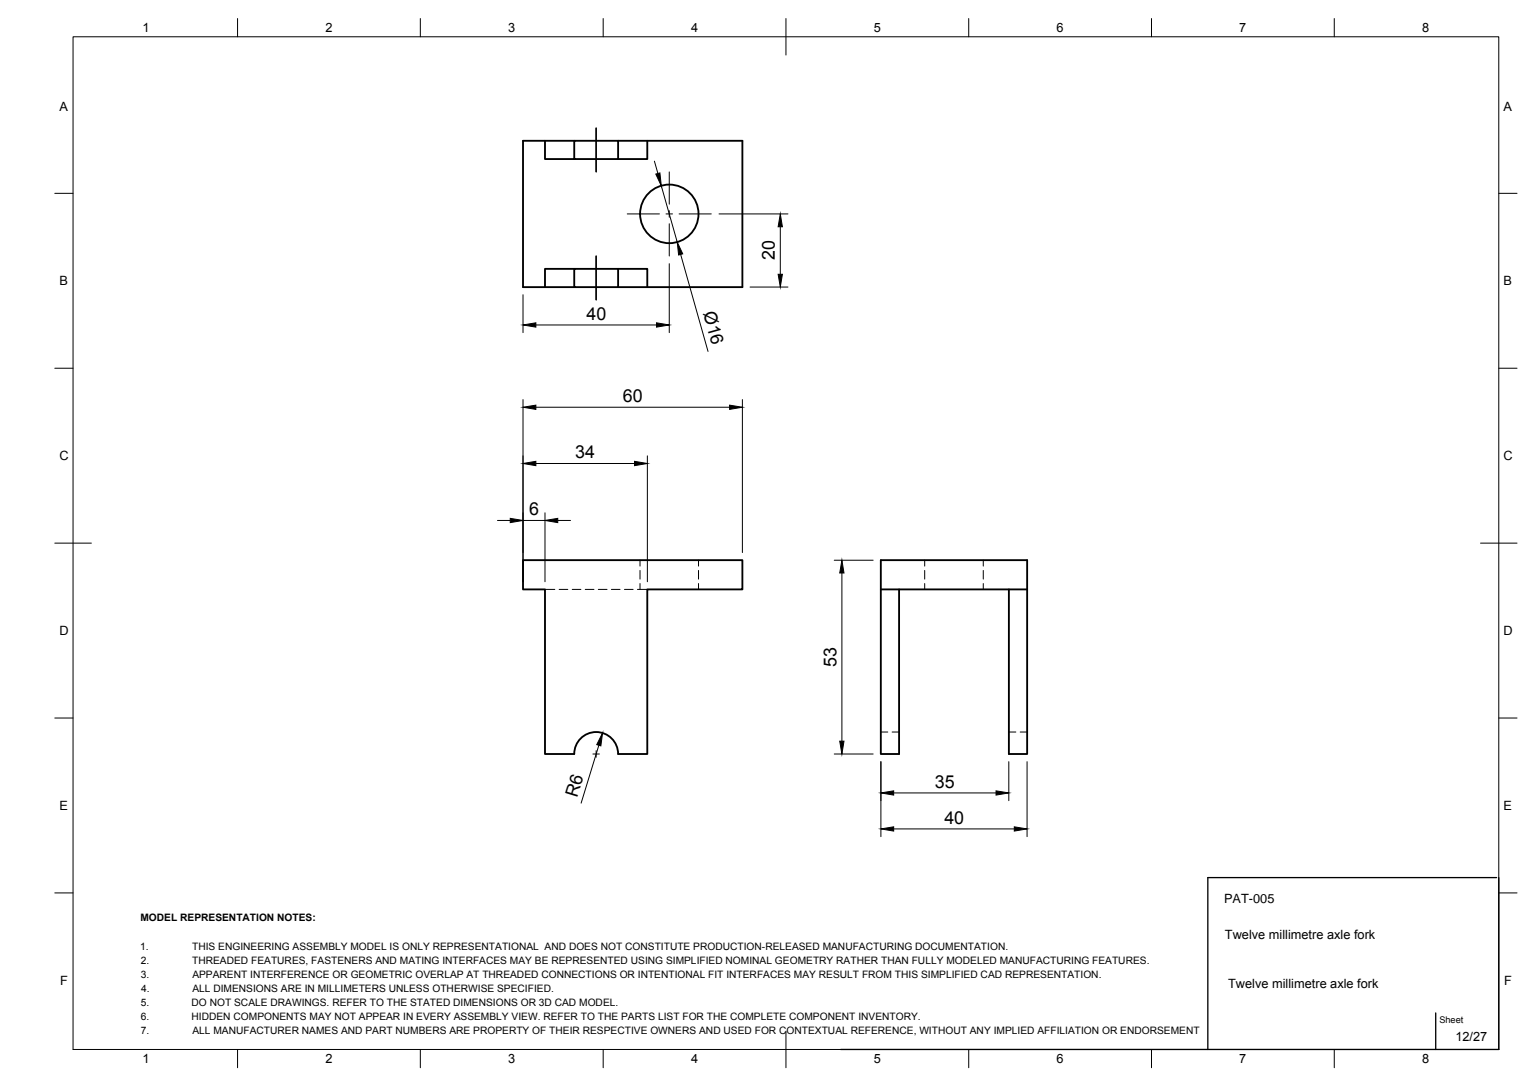
ISO-10303-21;
HEADER;
/* Generated by software containing ST-Developer
 * from STEP Tools, Inc. (www.steptools.com) 
 */

FILE_DESCRIPTION(
/* description */ ('Ball-race swivel caster'),
/* implementation_level */ '2;1');

FILE_NAME(
/* name */ 'Twelve millimetre axle fork.step',
/* time_stamp */ '2026-10-29T16:15:51-07:00',
/* author */ (''),
/* organization */ (''),
/* preprocessor_version */ 'ST-DEVELOPER v20.2',
/* originating_system */ 'Autodesk Translation Framework v15.17.0.0',
/* authorisation */ '');

FILE_SCHEMA (('AUTOMOTIVE_DESIGN { 1 0 10303 214 3 1 1 }'));
ENDSEC;

DATA;
#10=MECHANICAL_DESIGN_GEOMETRIC_PRESENTATION_REPRESENTATION('',(#314),#7816);
#265=SHAPE_REPRESENTATION_RELATIONSHIP('SRR','None',#7912,#285);
#285=ADVANCED_BREP_SHAPE_REPRESENTATION('',(#350),#7801);
#314=STYLED_ITEM('',(#8097),#350);
#350=MANIFOLD_SOLID_BREP('Body1',#3720);
#412=FACE_BOUND('',#883,.T.);
#413=FACE_BOUND('',#891,.T.);
#465=PLANE('',#4238);
#466=PLANE('',#4239);
#467=PLANE('',#4240);
#468=PLANE('',#4241);
#469=PLANE('',#4242);
#470=PLANE('',#4243);
#471=PLANE('',#4244);
#472=PLANE('',#4245);
#473=PLANE('',#4246);
#474=PLANE('',#4247);
#475=PLANE('',#4248);
#476=PLANE('',#4249);
#477=PLANE('',#4250);
#478=PLANE('',#4251);
#479=PLANE('',#4252);
#480=PLANE('',#4253);
#619=FACE_OUTER_BOUND('',#871,.T.);
#620=FACE_OUTER_BOUND('',#872,.T.);
#621=FACE_OUTER_BOUND('',#873,.T.);
#622=FACE_OUTER_BOUND('',#874,.T.);
#623=FACE_OUTER_BOUND('',#875,.T.);
#624=FACE_OUTER_BOUND('',#876,.T.);
#625=FACE_OUTER_BOUND('',#877,.T.);
#626=FACE_OUTER_BOUND('',#878,.T.);
#627=FACE_OUTER_BOUND('',#879,.T.);
#628=FACE_OUTER_BOUND('',#880,.T.);
#629=FACE_OUTER_BOUND('',#881,.T.);
#630=FACE_OUTER_BOUND('',#882,.T.);
#631=FACE_OUTER_BOUND('',#884,.T.);
#632=FACE_OUTER_BOUND('',#885,.T.);
#633=FACE_OUTER_BOUND('',#886,.T.);
#634=FACE_OUTER_BOUND('',#887,.T.);
#635=FACE_OUTER_BOUND('',#888,.T.);
#636=FACE_OUTER_BOUND('',#889,.T.);
#637=FACE_OUTER_BOUND('',#890,.T.);
#871=EDGE_LOOP('',(#2977,#2978,#2979,#2980));
#872=EDGE_LOOP('',(#2981,#2982,#2983,#2984));
#873=EDGE_LOOP('',(#2985,#2986,#2987,#2988));
#874=EDGE_LOOP('',(#2989,#2990,#2991,#2992,#2993,#2994,#2995,#2996,#2997,
#2998));
#875=EDGE_LOOP('',(#2999,#3000,#3001,#3002));
#876=EDGE_LOOP('',(#3003,#3004,#3005,#3006));
#877=EDGE_LOOP('',(#3007,#3008,#3009,#3010,#3011,#3012,#3013,#3014,#3015,
#3016));
#878=EDGE_LOOP('',(#3017,#3018,#3019,#3020));
#879=EDGE_LOOP('',(#3021,#3022,#3023,#3024));
#880=EDGE_LOOP('',(#3025,#3026,#3027,#3028));
#881=EDGE_LOOP('',(#3029,#3030,#3031,#3032,#3033,#3034));
#882=EDGE_LOOP('',(#3035,#3036,#3037,#3038,#3039,#3040,#3041,#3042,#3043,
#3044,#3045,#3046));
#883=EDGE_LOOP('',(#3047));
#884=EDGE_LOOP('',(#3048,#3049,#3050,#3051,#3052,#3053));
#885=EDGE_LOOP('',(#3054,#3055,#3056,#3057));
#886=EDGE_LOOP('',(#3058,#3059,#3060,#3061));
#887=EDGE_LOOP('',(#3062,#3063,#3064,#3065));
#888=EDGE_LOOP('',(#3066,#3067,#3068,#3069));
#889=EDGE_LOOP('',(#3070,#3071,#3072,#3073));
#890=EDGE_LOOP('',(#3074,#3075,#3076,#3077));
#891=EDGE_LOOP('',(#3078));
#1067=LINE('',#6943,#1222);
#1068=LINE('',#6950,#1223);
#1069=LINE('',#6953,#1224);
#1070=LINE('',#6957,#1225);
#1071=LINE('',#6961,#1226);
#1072=LINE('',#6965,#1227);
#1073=LINE('',#6967,#1228);
#1074=LINE('',#6969,#1229);
#1075=LINE('',#6971,#1230);
#1076=LINE('',#6973,#1231);
#1077=LINE('',#6975,#1232);
#1078=LINE('',#6977,#1233);
#1079=LINE('',#6979,#1234);
#1080=LINE('',#6980,#1235);
#1081=LINE('',#6983,#1236);
#1082=LINE('',#6984,#1237);
#1083=LINE('',#6987,#1238);
#1084=LINE('',#6988,#1239);
#1085=LINE('',#6991,#1240);
#1086=LINE('',#6993,#1241);
#1087=LINE('',#6995,#1242);
#1088=LINE('',#6997,#1243);
#1089=LINE('',#6999,#1244);
#1090=LINE('',#7001,#1245);
#1091=LINE('',#7003,#1246);
#1092=LINE('',#7005,#1247);
#1093=LINE('',#7006,#1248);
#1094=LINE('',#7009,#1249);
#1095=LINE('',#7010,#1250);
#1096=LINE('',#7013,#1251);
#1097=LINE('',#7014,#1252);
#1098=LINE('',#7017,#1253);
#1099=LINE('',#7018,#1254);
#1100=LINE('',#7020,#1255);
#1101=LINE('',#7022,#1256);
#1102=LINE('',#7024,#1257);
#1103=LINE('',#7026,#1258);
#1104=LINE('',#7027,#1259);
#1105=LINE('',#7028,#1260);
#1106=LINE('',#7031,#1261);
#1107=LINE('',#7032,#1262);
#1108=LINE('',#7033,#1263);
#1109=LINE('',#7036,#1264);
#1110=LINE('',#7039,#1265);
#1111=LINE('',#7041,#1266);
#1222=VECTOR('',#5083,0.8);
#1223=VECTOR('',#5090,1.);
#1224=VECTOR('',#5093,1.);
#1225=VECTOR('',#5096,1.);
#1226=VECTOR('',#5099,1.);
#1227=VECTOR('',#5104,1.);
#1228=VECTOR('',#5105,1.);
#1229=VECTOR('',#5106,1.);
#1230=VECTOR('',#5107,1.);
#1231=VECTOR('',#5108,1.);
#1232=VECTOR('',#5109,1.);
#1233=VECTOR('',#5110,1.);
#1234=VECTOR('',#5111,1.);
#1235=VECTOR('',#5112,1.);
#1236=VECTOR('',#5115,1.);
#1237=VECTOR('',#5116,1.);
#1238=VECTOR('',#5119,1.);
#1239=VECTOR('',#5120,1.);
#1240=VECTOR('',#5123,1.);
#1241=VECTOR('',#5124,1.);
#1242=VECTOR('',#5125,1.);
#1243=VECTOR('',#5126,1.);
#1244=VECTOR('',#5127,1.);
#1245=VECTOR('',#5128,1.);
#1246=VECTOR('',#5129,1.);
#1247=VECTOR('',#5130,1.);
#1248=VECTOR('',#5131,1.);
#1249=VECTOR('',#5134,1.);
#1250=VECTOR('',#5135,1.);
#1251=VECTOR('',#5138,1.);
#1252=VECTOR('',#5139,1.);
#1253=VECTOR('',#5142,1.);
#1254=VECTOR('',#5143,1.);
#1255=VECTOR('',#5146,1.);
#1256=VECTOR('',#5149,1.);
#1257=VECTOR('',#5150,1.);
#1258=VECTOR('',#5151,1.);
#1259=VECTOR('',#5152,1.);
#1260=VECTOR('',#5153,1.);
#1261=VECTOR('',#5156,1.);
#1262=VECTOR('',#5157,1.);
#1263=VECTOR('',#5158,1.);
#1264=VECTOR('',#5163,1.);
#1265=VECTOR('',#5168,1.);
#1266=VECTOR('',#5171,1.);
#1473=CIRCLE('',#4230,0.8);
#1474=CIRCLE('',#4231,0.8);
#1475=CIRCLE('',#4233,0.6);
#1476=CIRCLE('',#4234,0.6);
#1477=CIRCLE('',#4236,0.6);
#1478=CIRCLE('',#4237,0.6);
#1779=VERTEX_POINT('',#6940);
#1780=VERTEX_POINT('',#6942);
#1781=VERTEX_POINT('',#6946);
#1782=VERTEX_POINT('',#6947);
#1783=VERTEX_POINT('',#6949);
#1784=VERTEX_POINT('',#6951);
#1785=VERTEX_POINT('',#6955);
#1786=VERTEX_POINT('',#6956);
#1787=VERTEX_POINT('',#6958);
#1788=VERTEX_POINT('',#6960);
#1789=VERTEX_POINT('',#6964);
#1790=VERTEX_POINT('',#6966);
#1791=VERTEX_POINT('',#6968);
#1792=VERTEX_POINT('',#6970);
#1793=VERTEX_POINT('',#6972);
#1794=VERTEX_POINT('',#6974);
#1795=VERTEX_POINT('',#6976);
#1796=VERTEX_POINT('',#6978);
#1797=VERTEX_POINT('',#6982);
#1798=VERTEX_POINT('',#6986);
#1799=VERTEX_POINT('',#6990);
#1800=VERTEX_POINT('',#6992);
#1801=VERTEX_POINT('',#6994);
#1802=VERTEX_POINT('',#6996);
#1803=VERTEX_POINT('',#6998);
#1804=VERTEX_POINT('',#7000);
#1805=VERTEX_POINT('',#7002);
#1806=VERTEX_POINT('',#7004);
#1807=VERTEX_POINT('',#7008);
#1808=VERTEX_POINT('',#7012);
#1809=VERTEX_POINT('',#7016);
#1810=VERTEX_POINT('',#7023);
#1811=VERTEX_POINT('',#7025);
#1812=VERTEX_POINT('',#7030);
#2208=EDGE_CURVE('',#1779,#1779,#1473,.T.);
#2209=EDGE_CURVE('',#1779,#1780,#1067,.T.);
#2210=EDGE_CURVE('',#1780,#1780,#1474,.T.);
#2211=EDGE_CURVE('',#1781,#1782,#1475,.T.);
#2212=EDGE_CURVE('',#1783,#1781,#1068,.T.);
#2213=EDGE_CURVE('',#1784,#1783,#1476,.T.);
#2214=EDGE_CURVE('',#1782,#1784,#1069,.T.);
#2215=EDGE_CURVE('',#1785,#1786,#1070,.T.);
#2216=EDGE_CURVE('',#1787,#1785,#1477,.T.);
#2217=EDGE_CURVE('',#1788,#1787,#1071,.T.);
#2218=EDGE_CURVE('',#1786,#1788,#1478,.T.);
#2219=EDGE_CURVE('',#1785,#1789,#1072,.T.);
#2220=EDGE_CURVE('',#1789,#1790,#1073,.T.);
#2221=EDGE_CURVE('',#1790,#1791,#1074,.T.);
#2222=EDGE_CURVE('',#1791,#1792,#1075,.T.);
#2223=EDGE_CURVE('',#1793,#1792,#1076,.T.);
#2224=EDGE_CURVE('',#1794,#1793,#1077,.T.);
#2225=EDGE_CURVE('',#1794,#1795,#1078,.T.);
#2226=EDGE_CURVE('',#1795,#1796,#1079,.T.);
#2227=EDGE_CURVE('',#1796,#1787,#1080,.T.);
#2228=EDGE_CURVE('',#1797,#1786,#1081,.T.);
#2229=EDGE_CURVE('',#1797,#1789,#1082,.T.);
#2230=EDGE_CURVE('',#1798,#1796,#1083,.T.);
#2231=EDGE_CURVE('',#1788,#1798,#1084,.T.);
#2232=EDGE_CURVE('',#1783,#1799,#1085,.T.);
#2233=EDGE_CURVE('',#1799,#1800,#1086,.T.);
#2234=EDGE_CURVE('',#1800,#1801,#1087,.T.);
#2235=EDGE_CURVE('',#1801,#1802,#1088,.T.);
#2236=EDGE_CURVE('',#1803,#1802,#1089,.T.);
#2237=EDGE_CURVE('',#1804,#1803,#1090,.T.);
#2238=EDGE_CURVE('',#1804,#1805,#1091,.T.);
#2239=EDGE_CURVE('',#1805,#1806,#1092,.T.);
#2240=EDGE_CURVE('',#1806,#1784,#1093,.T.);
#2241=EDGE_CURVE('',#1807,#1781,#1094,.T.);
#2242=EDGE_CURVE('',#1799,#1807,#1095,.T.);
#2243=EDGE_CURVE('',#1790,#1808,#1096,.T.);
#2244=EDGE_CURVE('',#1808,#1797,#1097,.T.);
#2245=EDGE_CURVE('',#1809,#1795,#1098,.T.);
#2246=EDGE_CURVE('',#1798,#1809,#1099,.T.);
#2247=EDGE_CURVE('',#1808,#1809,#1100,.T.);
#2248=EDGE_CURVE('',#1801,#1794,#1101,.T.);
#2249=EDGE_CURVE('',#1800,#1810,#1102,.T.);
#2250=EDGE_CURVE('',#1810,#1811,#1103,.T.);
#2251=EDGE_CURVE('',#1811,#1805,#1104,.T.);
#2252=EDGE_CURVE('',#1791,#1804,#1105,.T.);
#2253=EDGE_CURVE('',#1782,#1812,#1106,.T.);
#2254=EDGE_CURVE('',#1812,#1811,#1107,.T.);
#2255=EDGE_CURVE('',#1810,#1807,#1108,.T.);
#2256=EDGE_CURVE('',#1806,#1812,#1109,.T.);
#2257=EDGE_CURVE('',#1802,#1793,#1110,.T.);
#2258=EDGE_CURVE('',#1792,#1803,#1111,.T.);
#2977=ORIENTED_EDGE('',*,*,#2208,.F.);
#2978=ORIENTED_EDGE('',*,*,#2209,.T.);
#2979=ORIENTED_EDGE('',*,*,#2210,.F.);
#2980=ORIENTED_EDGE('',*,*,#2209,.F.);
#2981=ORIENTED_EDGE('',*,*,#2211,.F.);
#2982=ORIENTED_EDGE('',*,*,#2212,.F.);
#2983=ORIENTED_EDGE('',*,*,#2213,.F.);
#2984=ORIENTED_EDGE('',*,*,#2214,.F.);
#2985=ORIENTED_EDGE('',*,*,#2215,.F.);
#2986=ORIENTED_EDGE('',*,*,#2216,.F.);
#2987=ORIENTED_EDGE('',*,*,#2217,.F.);
#2988=ORIENTED_EDGE('',*,*,#2218,.F.);
#2989=ORIENTED_EDGE('',*,*,#2216,.T.);
#2990=ORIENTED_EDGE('',*,*,#2219,.T.);
#2991=ORIENTED_EDGE('',*,*,#2220,.T.);
#2992=ORIENTED_EDGE('',*,*,#2221,.T.);
#2993=ORIENTED_EDGE('',*,*,#2222,.T.);
#2994=ORIENTED_EDGE('',*,*,#2223,.F.);
#2995=ORIENTED_EDGE('',*,*,#2224,.F.);
#2996=ORIENTED_EDGE('',*,*,#2225,.T.);
#2997=ORIENTED_EDGE('',*,*,#2226,.T.);
#2998=ORIENTED_EDGE('',*,*,#2227,.T.);
#2999=ORIENTED_EDGE('',*,*,#2215,.T.);
#3000=ORIENTED_EDGE('',*,*,#2228,.F.);
#3001=ORIENTED_EDGE('',*,*,#2229,.T.);
#3002=ORIENTED_EDGE('',*,*,#2219,.F.);
#3003=ORIENTED_EDGE('',*,*,#2217,.T.);
#3004=ORIENTED_EDGE('',*,*,#2227,.F.);
#3005=ORIENTED_EDGE('',*,*,#2230,.F.);
#3006=ORIENTED_EDGE('',*,*,#2231,.F.);
#3007=ORIENTED_EDGE('',*,*,#2213,.T.);
#3008=ORIENTED_EDGE('',*,*,#2232,.T.);
#3009=ORIENTED_EDGE('',*,*,#2233,.T.);
#3010=ORIENTED_EDGE('',*,*,#2234,.T.);
#3011=ORIENTED_EDGE('',*,*,#2235,.T.);
#3012=ORIENTED_EDGE('',*,*,#2236,.F.);
#3013=ORIENTED_EDGE('',*,*,#2237,.F.);
#3014=ORIENTED_EDGE('',*,*,#2238,.T.);
#3015=ORIENTED_EDGE('',*,*,#2239,.T.);
#3016=ORIENTED_EDGE('',*,*,#2240,.T.);
#3017=ORIENTED_EDGE('',*,*,#2212,.T.);
#3018=ORIENTED_EDGE('',*,*,#2241,.F.);
#3019=ORIENTED_EDGE('',*,*,#2242,.F.);
#3020=ORIENTED_EDGE('',*,*,#2232,.F.);
#3021=ORIENTED_EDGE('',*,*,#2243,.F.);
#3022=ORIENTED_EDGE('',*,*,#2220,.F.);
#3023=ORIENTED_EDGE('',*,*,#2229,.F.);
#3024=ORIENTED_EDGE('',*,*,#2244,.F.);
#3025=ORIENTED_EDGE('',*,*,#2245,.F.);
#3026=ORIENTED_EDGE('',*,*,#2246,.F.);
#3027=ORIENTED_EDGE('',*,*,#2230,.T.);
#3028=ORIENTED_EDGE('',*,*,#2226,.F.);
#3029=ORIENTED_EDGE('',*,*,#2218,.T.);
#3030=ORIENTED_EDGE('',*,*,#2231,.T.);
#3031=ORIENTED_EDGE('',*,*,#2246,.T.);
#3032=ORIENTED_EDGE('',*,*,#2247,.F.);
#3033=ORIENTED_EDGE('',*,*,#2244,.T.);
#3034=ORIENTED_EDGE('',*,*,#2228,.T.);
#3035=ORIENTED_EDGE('',*,*,#2243,.T.);
#3036=ORIENTED_EDGE('',*,*,#2247,.T.);
#3037=ORIENTED_EDGE('',*,*,#2245,.T.);
#3038=ORIENTED_EDGE('',*,*,#2225,.F.);
#3039=ORIENTED_EDGE('',*,*,#2248,.F.);
#3040=ORIENTED_EDGE('',*,*,#2234,.F.);
#3041=ORIENTED_EDGE('',*,*,#2249,.T.);
#3042=ORIENTED_EDGE('',*,*,#2250,.T.);
#3043=ORIENTED_EDGE('',*,*,#2251,.T.);
#3044=ORIENTED_EDGE('',*,*,#2238,.F.);
#3045=ORIENTED_EDGE('',*,*,#2252,.F.);
#3046=ORIENTED_EDGE('',*,*,#2221,.F.);
#3047=ORIENTED_EDGE('',*,*,#2208,.T.);
#3048=ORIENTED_EDGE('',*,*,#2211,.T.);
#3049=ORIENTED_EDGE('',*,*,#2253,.T.);
#3050=ORIENTED_EDGE('',*,*,#2254,.T.);
#3051=ORIENTED_EDGE('',*,*,#2250,.F.);
#3052=ORIENTED_EDGE('',*,*,#2255,.T.);
#3053=ORIENTED_EDGE('',*,*,#2241,.T.);
#3054=ORIENTED_EDGE('',*,*,#2249,.F.);
#3055=ORIENTED_EDGE('',*,*,#2233,.F.);
#3056=ORIENTED_EDGE('',*,*,#2242,.T.);
#3057=ORIENTED_EDGE('',*,*,#2255,.F.);
#3058=ORIENTED_EDGE('',*,*,#2251,.F.);
#3059=ORIENTED_EDGE('',*,*,#2254,.F.);
#3060=ORIENTED_EDGE('',*,*,#2256,.F.);
#3061=ORIENTED_EDGE('',*,*,#2239,.F.);
#3062=ORIENTED_EDGE('',*,*,#2214,.T.);
#3063=ORIENTED_EDGE('',*,*,#2240,.F.);
#3064=ORIENTED_EDGE('',*,*,#2256,.T.);
#3065=ORIENTED_EDGE('',*,*,#2253,.F.);
#3066=ORIENTED_EDGE('',*,*,#2248,.T.);
#3067=ORIENTED_EDGE('',*,*,#2224,.T.);
#3068=ORIENTED_EDGE('',*,*,#2257,.F.);
#3069=ORIENTED_EDGE('',*,*,#2235,.F.);
#3070=ORIENTED_EDGE('',*,*,#2252,.T.);
#3071=ORIENTED_EDGE('',*,*,#2237,.T.);
#3072=ORIENTED_EDGE('',*,*,#2258,.F.);
#3073=ORIENTED_EDGE('',*,*,#2222,.F.);
#3074=ORIENTED_EDGE('',*,*,#2258,.T.);
#3075=ORIENTED_EDGE('',*,*,#2236,.T.);
#3076=ORIENTED_EDGE('',*,*,#2257,.T.);
#3077=ORIENTED_EDGE('',*,*,#2223,.T.);
#3078=ORIENTED_EDGE('',*,*,#2210,.T.);
#3463=CYLINDRICAL_SURFACE('',#4229,0.8);
#3464=CYLINDRICAL_SURFACE('',#4232,0.6);
#3465=CYLINDRICAL_SURFACE('',#4235,0.6);
#3590=ADVANCED_FACE('',(#619),#3463,.F.);
#3591=ADVANCED_FACE('',(#620),#3464,.F.);
#3592=ADVANCED_FACE('',(#621),#3465,.F.);
#3593=ADVANCED_FACE('',(#622),#465,.T.);
#3594=ADVANCED_FACE('',(#623),#466,.T.);
#3595=ADVANCED_FACE('',(#624),#467,.T.);
#3596=ADVANCED_FACE('',(#625),#468,.T.);
#3597=ADVANCED_FACE('',(#626),#469,.T.);
#3598=ADVANCED_FACE('',(#627),#470,.T.);
#3599=ADVANCED_FACE('',(#628),#471,.T.);
#3600=ADVANCED_FACE('',(#629),#472,.F.);
#3601=ADVANCED_FACE('',(#630,#412),#473,.F.);
#3602=ADVANCED_FACE('',(#631),#474,.T.);
#3603=ADVANCED_FACE('',(#632),#475,.T.);
#3604=ADVANCED_FACE('',(#633),#476,.T.);
#3605=ADVANCED_FACE('',(#634),#477,.T.);
#3606=ADVANCED_FACE('',(#635),#478,.T.);
#3607=ADVANCED_FACE('',(#636),#479,.T.);
#3608=ADVANCED_FACE('',(#637,#413),#480,.T.);
#3720=CLOSED_SHELL('',(#3590,#3591,#3592,#3593,#3594,#3595,#3596,#3597,
#3598,#3599,#3600,#3601,#3602,#3603,#3604,#3605,#3606,#3607,#3608));
#4228=AXIS2_PLACEMENT_3D('',#6938,#5077,#5078);
#4229=AXIS2_PLACEMENT_3D('',#6939,#5079,#5080);
#4230=AXIS2_PLACEMENT_3D('',#6941,#5081,#5082);
#4231=AXIS2_PLACEMENT_3D('',#6944,#5084,#5085);
#4232=AXIS2_PLACEMENT_3D('',#6945,#5086,#5087);
#4233=AXIS2_PLACEMENT_3D('',#6948,#5088,#5089);
#4234=AXIS2_PLACEMENT_3D('',#6952,#5091,#5092);
#4235=AXIS2_PLACEMENT_3D('',#6954,#5094,#5095);
#4236=AXIS2_PLACEMENT_3D('',#6959,#5097,#5098);
#4237=AXIS2_PLACEMENT_3D('',#6962,#5100,#5101);
#4238=AXIS2_PLACEMENT_3D('',#6963,#5102,#5103);
#4239=AXIS2_PLACEMENT_3D('',#6981,#5113,#5114);
#4240=AXIS2_PLACEMENT_3D('',#6985,#5117,#5118);
#4241=AXIS2_PLACEMENT_3D('',#6989,#5121,#5122);
#4242=AXIS2_PLACEMENT_3D('',#7007,#5132,#5133);
#4243=AXIS2_PLACEMENT_3D('',#7011,#5136,#5137);
#4244=AXIS2_PLACEMENT_3D('',#7015,#5140,#5141);
#4245=AXIS2_PLACEMENT_3D('',#7019,#5144,#5145);
#4246=AXIS2_PLACEMENT_3D('',#7021,#5147,#5148);
#4247=AXIS2_PLACEMENT_3D('',#7029,#5154,#5155);
#4248=AXIS2_PLACEMENT_3D('',#7034,#5159,#5160);
#4249=AXIS2_PLACEMENT_3D('',#7035,#5161,#5162);
#4250=AXIS2_PLACEMENT_3D('',#7037,#5164,#5165);
#4251=AXIS2_PLACEMENT_3D('',#7038,#5166,#5167);
#4252=AXIS2_PLACEMENT_3D('',#7040,#5169,#5170);
#4253=AXIS2_PLACEMENT_3D('',#7042,#5172,#5173);
#5077=DIRECTION('axis',(0.,0.,1.));
#5078=DIRECTION('refdir',(1.,0.,0.));
#5079=DIRECTION('center_axis',(0.,0.,1.));
#5080=DIRECTION('ref_axis',(1.,0.,0.));
#5081=DIRECTION('center_axis',(0.,0.,1.));
#5082=DIRECTION('ref_axis',(1.,0.,0.));
#5083=DIRECTION('',(0.,0.,1.));
#5084=DIRECTION('center_axis',(0.,0.,-1.));
#5085=DIRECTION('ref_axis',(1.,0.,0.));
#5086=DIRECTION('center_axis',(0.,1.,0.));
#5087=DIRECTION('ref_axis',(1.,0.,0.));
#5088=DIRECTION('center_axis',(0.,-1.,0.));
#5089=DIRECTION('ref_axis',(1.,0.,0.));
#5090=DIRECTION('',(0.,1.,0.));
#5091=DIRECTION('center_axis',(0.,1.,0.));
#5092=DIRECTION('ref_axis',(1.,0.,0.));
#5093=DIRECTION('',(0.,-1.,0.));
#5094=DIRECTION('center_axis',(0.,1.,0.));
#5095=DIRECTION('ref_axis',(1.,0.,0.));
#5096=DIRECTION('',(0.,-1.,0.));
#5097=DIRECTION('center_axis',(0.,-1.,0.));
#5098=DIRECTION('ref_axis',(1.,0.,0.));
#5099=DIRECTION('',(0.,1.,0.));
#5100=DIRECTION('center_axis',(0.,1.,0.));
#5101=DIRECTION('ref_axis',(1.,0.,0.));
#5102=DIRECTION('center_axis',(0.,1.,0.));
#5103=DIRECTION('ref_axis',(-1.,0.,0.));
#5104=DIRECTION('',(-1.,0.,0.));
#5105=DIRECTION('',(0.,0.,1.));
#5106=DIRECTION('',(-1.,0.,0.));
#5107=DIRECTION('',(0.,0.,1.));
#5108=DIRECTION('',(-1.,0.,0.));
#5109=DIRECTION('',(0.,0.,1.));
#5110=DIRECTION('',(-1.,0.,0.));
#5111=DIRECTION('',(0.,0.,-1.));
#5112=DIRECTION('',(-1.,0.,0.));
#5113=DIRECTION('center_axis',(0.,0.,-1.));
#5114=DIRECTION('ref_axis',(-1.,0.,0.));
#5115=DIRECTION('',(1.,0.,0.));
#5116=DIRECTION('',(0.,1.,0.));
#5117=DIRECTION('center_axis',(0.,0.,-1.));
#5118=DIRECTION('ref_axis',(-1.,0.,0.));
#5119=DIRECTION('',(0.,1.,0.));
#5120=DIRECTION('',(1.,0.,0.));
#5121=DIRECTION('center_axis',(0.,-1.,0.));
#5122=DIRECTION('ref_axis',(1.,0.,0.));
#5123=DIRECTION('',(1.,0.,0.));
#5124=DIRECTION('',(0.,0.,1.));
#5125=DIRECTION('',(1.,0.,0.));
#5126=DIRECTION('',(0.,0.,1.));
#5127=DIRECTION('',(1.,0.,0.));
#5128=DIRECTION('',(0.,0.,1.));
#5129=DIRECTION('',(1.,0.,0.));
#5130=DIRECTION('',(0.,0.,-1.));
#5131=DIRECTION('',(1.,0.,0.));
#5132=DIRECTION('center_axis',(0.,0.,-1.));
#5133=DIRECTION('ref_axis',(-1.,0.,0.));
#5134=DIRECTION('',(-1.,0.,0.));
#5135=DIRECTION('',(0.,1.,0.));
#5136=DIRECTION('center_axis',(-1.,0.,0.));
#5137=DIRECTION('ref_axis',(0.,0.,1.));
#5138=DIRECTION('',(0.,-1.,0.));
#5139=DIRECTION('',(0.,0.,-1.));
#5140=DIRECTION('center_axis',(1.,0.,0.));
#5141=DIRECTION('ref_axis',(0.,0.,-1.));
#5142=DIRECTION('',(0.,1.,0.));
#5143=DIRECTION('',(0.,0.,1.));
#5144=DIRECTION('center_axis',(0.,1.,0.));
#5145=DIRECTION('ref_axis',(1.,0.,0.));
#5146=DIRECTION('',(1.,0.,0.));
#5147=DIRECTION('center_axis',(0.,0.,1.));
#5148=DIRECTION('ref_axis',(1.,0.,0.));
#5149=DIRECTION('',(0.,1.,0.));
#5150=DIRECTION('',(0.,1.,0.));
#5151=DIRECTION('',(-1.,0.,0.));
#5152=DIRECTION('',(0.,-1.,0.));
#5153=DIRECTION('',(0.,-1.,0.));
#5154=DIRECTION('center_axis',(0.,1.,0.));
#5155=DIRECTION('ref_axis',(0.,0.,1.));
#5156=DIRECTION('',(-1.,0.,0.));
#5157=DIRECTION('',(0.,0.,1.));
#5158=DIRECTION('',(0.,0.,-1.));
#5159=DIRECTION('center_axis',(1.,0.,0.));
#5160=DIRECTION('ref_axis',(0.,0.,-1.));
#5161=DIRECTION('center_axis',(-1.,0.,0.));
#5162=DIRECTION('ref_axis',(0.,0.,1.));
#5163=DIRECTION('',(0.,1.,0.));
#5164=DIRECTION('center_axis',(0.,0.,-1.));
#5165=DIRECTION('ref_axis',(-1.,0.,0.));
#5166=DIRECTION('center_axis',(1.,0.,0.));
#5167=DIRECTION('ref_axis',(0.,1.,0.));
#5168=DIRECTION('',(0.,1.,0.));
#5169=DIRECTION('center_axis',(-1.,0.,0.));
#5170=DIRECTION('ref_axis',(0.,-1.,0.));
#5171=DIRECTION('',(0.,-1.,0.));
#5172=DIRECTION('center_axis',(0.,0.,1.));
#5173=DIRECTION('ref_axis',(1.,0.,0.));
#6938=CARTESIAN_POINT('',(0.,0.,0.));
#6939=CARTESIAN_POINT('Origin',(-2.,0.,8.4));
#6940=CARTESIAN_POINT('',(-2.8,-9.79717439317883E-17,8.5));
#6941=CARTESIAN_POINT('Origin',(-2.,0.,8.5));
#6942=CARTESIAN_POINT('',(-2.8,9.79717439317883E-17,9.3));
#6943=CARTESIAN_POINT('',(-2.8,-9.79717439317883E-17,8.4));
#6944=CARTESIAN_POINT('Origin',(-2.,0.,9.3));
#6945=CARTESIAN_POINT('Origin',(0.,-2.1,4.));
#6946=CARTESIAN_POINT('',(0.6,-1.5,4.));
#6947=CARTESIAN_POINT('',(-0.6,-1.5,4.));
#6948=CARTESIAN_POINT('Origin',(0.,-1.5,4.));
#6949=CARTESIAN_POINT('',(0.6,-2.,4.));
#6950=CARTESIAN_POINT('',(0.6,-2.1,4.));
#6951=CARTESIAN_POINT('',(-0.6,-2.,4.));
#6952=CARTESIAN_POINT('Origin',(0.,-2.,4.));
#6953=CARTESIAN_POINT('',(-0.6,-2.1,4.));
#6954=CARTESIAN_POINT('Origin',(0.,-2.1,4.));
#6955=CARTESIAN_POINT('',(-0.6,2.,4.));
#6956=CARTESIAN_POINT('',(-0.6,1.5,4.));
#6957=CARTESIAN_POINT('',(-0.6,-2.1,4.));
#6958=CARTESIAN_POINT('',(0.6,2.,4.));
#6959=CARTESIAN_POINT('Origin',(0.,2.,4.));
#6960=CARTESIAN_POINT('',(0.6,1.5,4.));
#6961=CARTESIAN_POINT('',(0.6,-2.1,4.));
#6962=CARTESIAN_POINT('Origin',(0.,1.5,4.));
#6963=CARTESIAN_POINT('Origin',(2.,2.,8.5));
#6964=CARTESIAN_POINT('',(-1.4,2.,4.));
#6965=CARTESIAN_POINT('',(-1.4,2.,4.));
#6966=CARTESIAN_POINT('',(-1.4,2.,8.5));
#6967=CARTESIAN_POINT('',(-1.4,2.,8.9));
#6968=CARTESIAN_POINT('',(-4.,2.,8.5));
#6969=CARTESIAN_POINT('',(2.,2.,8.5));
#6970=CARTESIAN_POINT('',(-4.,2.,9.3));
#6971=CARTESIAN_POINT('',(-4.,2.,8.5));
#6972=CARTESIAN_POINT('',(2.,2.,9.3));
#6973=CARTESIAN_POINT('',(2.,2.,9.3));
#6974=CARTESIAN_POINT('',(2.,2.,8.5));
#6975=CARTESIAN_POINT('',(2.,2.,8.5));
#6976=CARTESIAN_POINT('',(1.4,2.,8.5));
#6977=CARTESIAN_POINT('',(2.,2.,8.5));
#6978=CARTESIAN_POINT('',(1.4,2.,4.));
#6979=CARTESIAN_POINT('',(1.4,2.,4.));
#6980=CARTESIAN_POINT('',(-1.4,2.,4.));
#6981=CARTESIAN_POINT('Origin',(1.4,1.5,4.));
#6982=CARTESIAN_POINT('',(-1.4,1.5,4.));
#6983=CARTESIAN_POINT('',(-1.4,1.5,4.));
#6984=CARTESIAN_POINT('',(-1.4,1.5,4.));
#6985=CARTESIAN_POINT('Origin',(1.4,1.5,4.));
#6986=CARTESIAN_POINT('',(1.4,1.5,4.));
#6987=CARTESIAN_POINT('',(1.4,1.5,4.));
#6988=CARTESIAN_POINT('',(-1.4,1.5,4.));
#6989=CARTESIAN_POINT('Origin',(-4.,-2.,8.5));
#6990=CARTESIAN_POINT('',(1.4,-2.,4.));
#6991=CARTESIAN_POINT('',(-1.4,-2.,4.));
#6992=CARTESIAN_POINT('',(1.4,-2.,8.5));
#6993=CARTESIAN_POINT('',(1.4,-2.,4.));
#6994=CARTESIAN_POINT('',(2.,-2.,8.5));
#6995=CARTESIAN_POINT('',(-4.,-2.,8.5));
#6996=CARTESIAN_POINT('',(2.,-2.,9.3));
#6997=CARTESIAN_POINT('',(2.,-2.,8.5));
#6998=CARTESIAN_POINT('',(-4.,-2.,9.3));
#6999=CARTESIAN_POINT('',(-4.,-2.,9.3));
#7000=CARTESIAN_POINT('',(-4.,-2.,8.5));
#7001=CARTESIAN_POINT('',(-4.,-2.,8.5));
#7002=CARTESIAN_POINT('',(-1.4,-2.,8.5));
#7003=CARTESIAN_POINT('',(-4.,-2.,8.5));
#7004=CARTESIAN_POINT('',(-1.4,-2.,4.));
#7005=CARTESIAN_POINT('',(-1.4,-2.,8.9));
#7006=CARTESIAN_POINT('',(-1.4,-2.,4.));
#7007=CARTESIAN_POINT('Origin',(1.4,-2.,4.));
#7008=CARTESIAN_POINT('',(1.4,-1.5,4.));
#7009=CARTESIAN_POINT('',(-1.4,-1.5,4.));
#7010=CARTESIAN_POINT('',(1.4,-2.,4.));
#7011=CARTESIAN_POINT('Origin',(-1.4,1.5,4.));
#7012=CARTESIAN_POINT('',(-1.4,1.5,8.5));
#7013=CARTESIAN_POINT('',(-1.4,0.75,8.5));
#7014=CARTESIAN_POINT('',(-1.4,1.5,8.9));
#7015=CARTESIAN_POINT('Origin',(1.4,1.5,8.9));
#7016=CARTESIAN_POINT('',(1.4,1.5,8.5));
#7017=CARTESIAN_POINT('',(1.4,0.75,8.5));
#7018=CARTESIAN_POINT('',(1.4,1.5,4.));
#7019=CARTESIAN_POINT('Origin',(0.,1.5,6.45));
#7020=CARTESIAN_POINT('',(-0.5,1.5,8.5));
#7021=CARTESIAN_POINT('Origin',(-1.,0.,8.5));
#7022=CARTESIAN_POINT('',(2.,-2.,8.5));
#7023=CARTESIAN_POINT('',(1.4,-1.5,8.5));
#7024=CARTESIAN_POINT('',(1.4,-1.,8.5));
#7025=CARTESIAN_POINT('',(-1.4,-1.5,8.5));
#7026=CARTESIAN_POINT('',(-0.5,-1.5,8.5));
#7027=CARTESIAN_POINT('',(-1.4,-1.,8.5));
#7028=CARTESIAN_POINT('',(-4.,2.,8.5));
#7029=CARTESIAN_POINT('Origin',(0.,-1.5,6.45));
#7030=CARTESIAN_POINT('',(-1.4,-1.5,4.));
#7031=CARTESIAN_POINT('',(-1.4,-1.5,4.));
#7032=CARTESIAN_POINT('',(-1.4,-1.5,8.9));
#7033=CARTESIAN_POINT('',(1.4,-1.5,4.));
#7034=CARTESIAN_POINT('Origin',(1.4,-2.,8.9));
#7035=CARTESIAN_POINT('Origin',(-1.4,-2.,4.));
#7036=CARTESIAN_POINT('',(-1.4,-2.,4.));
#7037=CARTESIAN_POINT('Origin',(1.4,-2.,4.));
#7038=CARTESIAN_POINT('Origin',(2.,-2.,8.5));
#7039=CARTESIAN_POINT('',(2.,-2.,9.3));
#7040=CARTESIAN_POINT('Origin',(-4.,2.,8.5));
#7041=CARTESIAN_POINT('',(-4.,2.,9.3));
#7042=CARTESIAN_POINT('Origin',(-1.,0.,9.3));
#7774=UNCERTAINTY_MEASURE_WITH_UNIT(LENGTH_MEASURE(0.001),#7817,
'DISTANCE_ACCURACY_VALUE',
'Maximum model space distance between geometric entities at asserted c
onnectivities');
#7789=UNCERTAINTY_MEASURE_WITH_UNIT(LENGTH_MEASURE(0.001),#7817,
'DISTANCE_ACCURACY_VALUE',
'Maximum model space distance between geometric entities at asserted c
onnectivities');
#7801=(
GEOMETRIC_REPRESENTATION_CONTEXT(3)
GLOBAL_UNCERTAINTY_ASSIGNED_CONTEXT((#7774))
GLOBAL_UNIT_ASSIGNED_CONTEXT((#7817,#7819,#7820))
REPRESENTATION_CONTEXT('','3D')
);
#7816=(
GEOMETRIC_REPRESENTATION_CONTEXT(3)
GLOBAL_UNCERTAINTY_ASSIGNED_CONTEXT((#7789))
GLOBAL_UNIT_ASSIGNED_CONTEXT((#7817,#7819,#7820))
REPRESENTATION_CONTEXT('','3D')
);
#7817=(
LENGTH_UNIT()
NAMED_UNIT(*)
SI_UNIT(.CENTI.,.METRE.)
);
#7819=(
NAMED_UNIT(*)
PLANE_ANGLE_UNIT()
SI_UNIT($,.RADIAN.)
);
#7820=(
NAMED_UNIT(*)
SI_UNIT($,.STERADIAN.)
SOLID_ANGLE_UNIT()
);
#7832=SHAPE_DEFINITION_REPRESENTATION(#7866,#7912);
#7866=PRODUCT_DEFINITION_SHAPE('',$,#7939);
#7912=SHAPE_REPRESENTATION('',(#4228),#7801);
#7927=PRODUCT_DEFINITION_CONTEXT('part definition',#8007,'design');
#7939=PRODUCT_DEFINITION('Twelve millimetre axle fork',
'Twelve millimetre axle fork',#7965,#7927);
#7965=PRODUCT_DEFINITION_FORMATION('',$,#8020);
#8007=APPLICATION_CONTEXT(
'Core Data for Automotive Mechanical Design Process');
#8008=PRODUCT_CONTEXT('part definition',#8007,'mechanical');
#8020=PRODUCT('Twelve millimetre axle fork',
'Twelve millimetre axle fork','Twelve millimetre axle fork',(#8008));
#8091=COLOUR_RGB('Grey',0.48,0.52,0.57);
#8092=FILL_AREA_STYLE_COLOUR('',#8091);
#8093=FILL_AREA_STYLE('',(#8092));
#8094=SURFACE_STYLE_FILL_AREA(#8093);
#8095=SURFACE_SIDE_STYLE('',(#8094));
#8096=SURFACE_STYLE_USAGE(.BOTH.,#8095);
#8097=PRESENTATION_STYLE_ASSIGNMENT((#8096));
ENDSEC;
END-ISO-10303-21;
